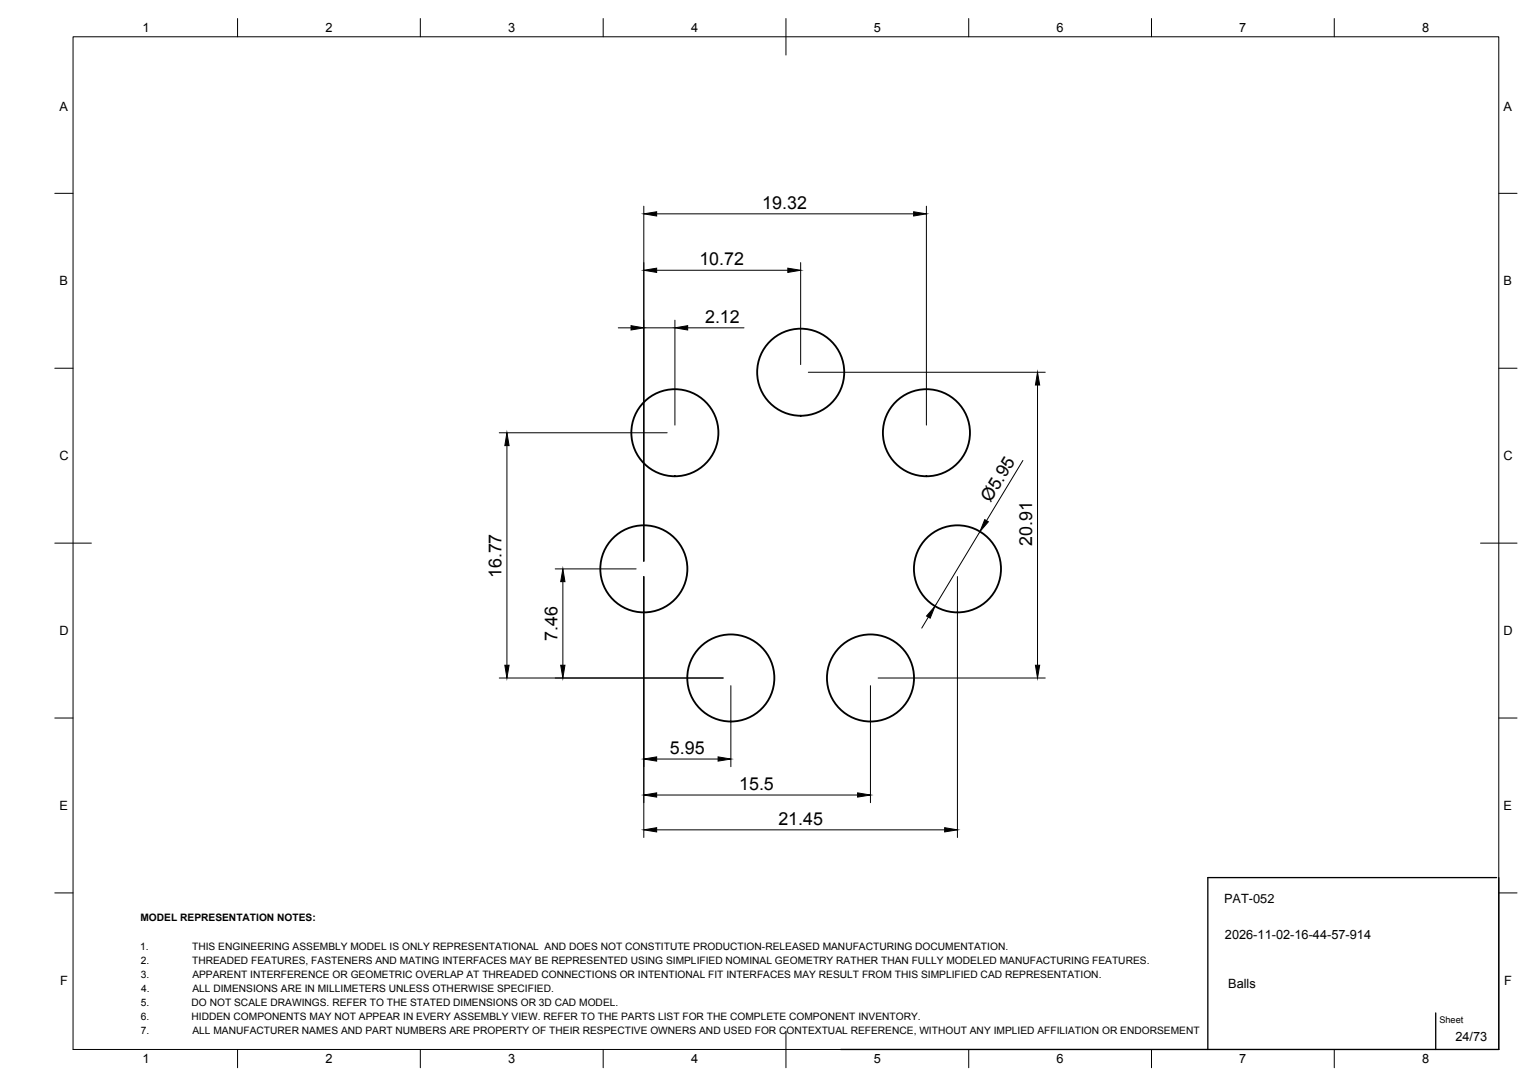
ISO-10303-21;
HEADER;
/* Generated by software containing ST-Developer
 * from STEP Tools, Inc. (www.steptools.com) 
 */

FILE_DESCRIPTION(
/* description */ ('Hand-crank gear train demonstrator'),
/* implementation_level */ '2;1');

FILE_NAME(
/* name */ 'Balls.step',
/* time_stamp */ '2026-10-28T03:22:13-07:00',
/* author */ (''),
/* organization */ (''),
/* preprocessor_version */ 'ST-DEVELOPER v20.2',
/* originating_system */ 'Autodesk Translation Framework v15.17.0.0',
/* authorisation */ '');

FILE_SCHEMA (('AUTOMOTIVE_DESIGN { 1 0 10303 214 3 1 1 }'));
ENDSEC;

DATA;
#10=MECHANICAL_DESIGN_GEOMETRIC_PRESENTATION_REPRESENTATION('',(#1202,#1203,#1204,#1205,#1206,#1207,#1208),#62758);
#991=SPHERICAL_SURFACE('',#17526,0.29765);
#992=SPHERICAL_SURFACE('',#17528,0.29765);
#993=SPHERICAL_SURFACE('',#17530,0.29765);
#994=SPHERICAL_SURFACE('',#17532,0.29765);
#995=SPHERICAL_SURFACE('',#17534,0.29765);
#996=SPHERICAL_SURFACE('',#17536,0.29765);
#997=SPHERICAL_SURFACE('',#17538,0.29765);
#1074=SHAPE_REPRESENTATION_RELATIONSHIP('SRR','None',#63047,#1138);
#1138=ADVANCED_BREP_SHAPE_REPRESENTATION('',(#1280,#1281,#1282,#1283,#1284,
#1285,#1286),#62701);
#1202=STYLED_ITEM('',(#63462),#1280);
#1203=STYLED_ITEM('',(#63462),#1281);
#1204=STYLED_ITEM('',(#63462),#1282);
#1205=STYLED_ITEM('',(#63462),#1283);
#1206=STYLED_ITEM('',(#63462),#1284);
#1207=STYLED_ITEM('',(#63462),#1285);
#1208=STYLED_ITEM('',(#63462),#1286);
#1280=MANIFOLD_SOLID_BREP('Body1',#16383);
#1281=MANIFOLD_SOLID_BREP('Body2',#16384);
#1282=MANIFOLD_SOLID_BREP('Body3',#16385);
#1283=MANIFOLD_SOLID_BREP('Body4',#16386);
#1284=MANIFOLD_SOLID_BREP('Body5',#16387);
#1285=MANIFOLD_SOLID_BREP('Body6',#16388);
#1286=MANIFOLD_SOLID_BREP('Body7',#16389);
#2277=FACE_OUTER_BOUND('',#3362,.T.);
#2278=FACE_OUTER_BOUND('',#3363,.T.);
#2279=FACE_OUTER_BOUND('',#3364,.T.);
#2280=FACE_OUTER_BOUND('',#3365,.T.);
#2281=FACE_OUTER_BOUND('',#3366,.T.);
#2282=FACE_OUTER_BOUND('',#3367,.T.);
#2283=FACE_OUTER_BOUND('',#3368,.T.);
#3362=EDGE_LOOP('',(#11523,#11524));
#3363=EDGE_LOOP('',(#11525,#11526));
#3364=EDGE_LOOP('',(#11527,#11528));
#3365=EDGE_LOOP('',(#11529,#11530));
#3366=EDGE_LOOP('',(#11531,#11532));
#3367=EDGE_LOOP('',(#11533,#11534));
#3368=EDGE_LOOP('',(#11535,#11536));
#6747=CIRCLE('',#17527,0.29765);
#6748=CIRCLE('',#17529,0.29765);
#6749=CIRCLE('',#17531,0.29765);
#6750=CIRCLE('',#17533,0.29765);
#6751=CIRCLE('',#17535,0.29765);
#6752=CIRCLE('',#17537,0.29765);
#6753=CIRCLE('',#17539,0.29765);
#7439=VERTEX_POINT('',#24052);
#7440=VERTEX_POINT('',#24053);
#7441=VERTEX_POINT('',#24056);
#7442=VERTEX_POINT('',#24057);
#7443=VERTEX_POINT('',#24060);
#7444=VERTEX_POINT('',#24061);
#7445=VERTEX_POINT('',#24064);
#7446=VERTEX_POINT('',#24065);
#7447=VERTEX_POINT('',#24068);
#7448=VERTEX_POINT('',#24069);
#7449=VERTEX_POINT('',#24072);
#7450=VERTEX_POINT('',#24073);
#7451=VERTEX_POINT('',#24076);
#7452=VERTEX_POINT('',#24077);
#9013=EDGE_CURVE('',#7439,#7440,#6747,.T.);
#9014=EDGE_CURVE('',#7441,#7442,#6748,.T.);
#9015=EDGE_CURVE('',#7443,#7444,#6749,.T.);
#9016=EDGE_CURVE('',#7445,#7446,#6750,.T.);
#9017=EDGE_CURVE('',#7447,#7448,#6751,.T.);
#9018=EDGE_CURVE('',#7449,#7450,#6752,.T.);
#9019=EDGE_CURVE('',#7451,#7452,#6753,.T.);
#11523=ORIENTED_EDGE('',*,*,#9013,.T.);
#11524=ORIENTED_EDGE('',*,*,#9013,.F.);
#11525=ORIENTED_EDGE('',*,*,#9014,.T.);
#11526=ORIENTED_EDGE('',*,*,#9014,.F.);
#11527=ORIENTED_EDGE('',*,*,#9015,.T.);
#11528=ORIENTED_EDGE('',*,*,#9015,.F.);
#11529=ORIENTED_EDGE('',*,*,#9016,.T.);
#11530=ORIENTED_EDGE('',*,*,#9016,.F.);
#11531=ORIENTED_EDGE('',*,*,#9017,.T.);
#11532=ORIENTED_EDGE('',*,*,#9017,.F.);
#11533=ORIENTED_EDGE('',*,*,#9018,.T.);
#11534=ORIENTED_EDGE('',*,*,#9018,.F.);
#11535=ORIENTED_EDGE('',*,*,#9019,.T.);
#11536=ORIENTED_EDGE('',*,*,#9019,.F.);
#15587=ADVANCED_FACE('',(#2277),#991,.T.);
#15588=ADVANCED_FACE('',(#2278),#992,.T.);
#15589=ADVANCED_FACE('',(#2279),#993,.T.);
#15590=ADVANCED_FACE('',(#2280),#994,.T.);
#15591=ADVANCED_FACE('',(#2281),#995,.T.);
#15592=ADVANCED_FACE('',(#2282),#996,.T.);
#15593=ADVANCED_FACE('',(#2283),#997,.T.);
#16383=CLOSED_SHELL('',(#15587));
#16384=CLOSED_SHELL('',(#15588));
#16385=CLOSED_SHELL('',(#15589));
#16386=CLOSED_SHELL('',(#15590));
#16387=CLOSED_SHELL('',(#15591));
#16388=CLOSED_SHELL('',(#15592));
#16389=CLOSED_SHELL('',(#15593));
#17525=AXIS2_PLACEMENT_3D('',#24050,#19712,#19713);
#17526=AXIS2_PLACEMENT_3D('',#24051,#19714,#19715);
#17527=AXIS2_PLACEMENT_3D('',#24054,#19716,#19717);
#17528=AXIS2_PLACEMENT_3D('',#24055,#19718,#19719);
#17529=AXIS2_PLACEMENT_3D('',#24058,#19720,#19721);
#17530=AXIS2_PLACEMENT_3D('',#24059,#19722,#19723);
#17531=AXIS2_PLACEMENT_3D('',#24062,#19724,#19725);
#17532=AXIS2_PLACEMENT_3D('',#24063,#19726,#19727);
#17533=AXIS2_PLACEMENT_3D('',#24066,#19728,#19729);
#17534=AXIS2_PLACEMENT_3D('',#24067,#19730,#19731);
#17535=AXIS2_PLACEMENT_3D('',#24070,#19732,#19733);
#17536=AXIS2_PLACEMENT_3D('',#24071,#19734,#19735);
#17537=AXIS2_PLACEMENT_3D('',#24074,#19736,#19737);
#17538=AXIS2_PLACEMENT_3D('',#24075,#19738,#19739);
#17539=AXIS2_PLACEMENT_3D('',#24078,#19740,#19741);
#19712=DIRECTION('axis',(0.,0.,1.));
#19713=DIRECTION('refdir',(1.,0.,0.));
#19714=DIRECTION('center_axis',(0.,0.,1.));
#19715=DIRECTION('ref_axis',(1.,0.,0.));
#19716=DIRECTION('center_axis',(1.22464679914735E-16,-1.,0.));
#19717=DIRECTION('ref_axis',(-1.,-1.22464679914735E-16,0.));
#19718=DIRECTION('center_axis',(0.78183148246803,0.,0.623489801858733));
#19719=DIRECTION('ref_axis',(0.623489801858734,0.,-0.78183148246803));
#19720=DIRECTION('center_axis',(7.63554790147315E-17,-1.,-9.57467422477103E-17));
#19721=DIRECTION('ref_axis',(-0.623489801858734,-1.22464679914735E-16,0.78183148246803));
#19722=DIRECTION('center_axis',(0.974927912181824,0.,-0.222520933956314));
#19723=DIRECTION('ref_axis',(-0.222520933956314,0.,-0.974927912181824));
#19724=DIRECTION('center_axis',(-2.7250954951288E-17,-1.,-1.19394234705288E-16));
#19725=DIRECTION('ref_axis',(0.222520933956314,-1.22464679914735E-16,0.974927912181824));
#19726=DIRECTION('center_axis',(0.433883739117558,0.,-0.900968867902419));
#19727=DIRECTION('ref_axis',(-0.900968867902419,0.,-0.433883739117558));
#19728=DIRECTION('center_axis',(-1.10336864020811E-16,-1.,-5.31354332312403E-17));
#19729=DIRECTION('ref_axis',(0.900968867902419,-1.22464679914735E-16,0.433883739117558));
#19730=DIRECTION('center_axis',(-0.433883739117558,0.,-0.900968867902419));
#19731=DIRECTION('ref_axis',(-0.900968867902419,0.,0.433883739117558));
#19732=DIRECTION('center_axis',(-1.10336864020811E-16,-1.,5.31354332312403E-17));
#19733=DIRECTION('ref_axis',(0.900968867902419,-1.22464679914735E-16,-0.433883739117558));
#19734=DIRECTION('center_axis',(-0.974927912181824,0.,-0.222520933956314));
#19735=DIRECTION('ref_axis',(-0.222520933956315,0.,0.974927912181824));
#19736=DIRECTION('center_axis',(-2.7250954951288E-17,-1.,1.19394234705288E-16));
#19737=DIRECTION('ref_axis',(0.222520933956315,-1.22464679914735E-16,-0.974927912181824));
#19738=DIRECTION('center_axis',(-0.78183148246803,0.,0.623489801858734));
#19739=DIRECTION('ref_axis',(0.623489801858733,0.,0.78183148246803));
#19740=DIRECTION('center_axis',(7.63554790147315E-17,-1.,9.57467422477103E-17));
#19741=DIRECTION('ref_axis',(-0.623489801858733,-1.22464679914735E-16,-0.78183148246803));
#24050=CARTESIAN_POINT('',(0.,0.,0.));
#24051=CARTESIAN_POINT('Origin',(1.1,0.,0.));
#24052=CARTESIAN_POINT('',(1.1,-2.23201749654651E-33,0.29765));
#24053=CARTESIAN_POINT('',(1.1,-2.23201749654651E-33,-0.29765));
#24054=CARTESIAN_POINT('Origin',(1.1,0.,0.));
#24055=CARTESIAN_POINT('Origin',(0.685838782044607,0.,-0.860014630714833));
#24056=CARTESIAN_POINT('',(0.918550922801216,-5.31350540756609E-33,-0.674432891191581));
#24057=CARTESIAN_POINT('',(0.453126641287998,8.49470414473068E-34,-1.04559637023808));
#24058=CARTESIAN_POINT('Origin',(0.685838782044607,0.,-0.860014630714833));
#24059=CARTESIAN_POINT('Origin',(-0.244773027351946,0.,-1.07242070340001));
#24060=CARTESIAN_POINT('',(0.0454142657089739,-2.23201749654651E-33,-1.1386540593921));
#24061=CARTESIAN_POINT('',(-0.534960320412865,-2.23201749654651E-33,-1.00618734740791));
#24062=CARTESIAN_POINT('Origin',(-0.244773027351946,0.,-1.07242070340001));
#24063=CARTESIAN_POINT('Origin',(-0.991065754692661,0.,-0.477272113029314));
#24064=CARTESIAN_POINT('',(-0.86192025974432,8.49470414473067E-34,-0.745445496560469));
#24065=CARTESIAN_POINT('',(-1.120211249641,-5.31350540756609E-33,-0.209098729498159));
#24066=CARTESIAN_POINT('Origin',(-0.991065754692661,0.,-0.477272113029314));
#24067=CARTESIAN_POINT('Origin',(-0.991065754692661,0.,0.477272113029314));
#24068=CARTESIAN_POINT('',(-1.120211249641,-2.23201749654651E-33,0.209098729498159));
#24069=CARTESIAN_POINT('',(-0.86192025974432,-2.23201749654651E-33,0.745445496560469));
#24070=CARTESIAN_POINT('Origin',(-0.991065754692661,0.,0.477272113029314));
#24071=CARTESIAN_POINT('Origin',(-0.244773027351946,0.,1.07242070340001));
#24072=CARTESIAN_POINT('',(-0.534960320412866,-2.23201749654651E-33,1.00618734740791));
#24073=CARTESIAN_POINT('',(0.0454142657089737,-2.23201749654651E-33,1.1386540593921));
#24074=CARTESIAN_POINT('Origin',(-0.244773027351946,0.,1.07242070340001));
#24075=CARTESIAN_POINT('Origin',(0.685838782044607,0.,0.860014630714833));
#24076=CARTESIAN_POINT('',(0.453126641287998,-2.23201749654651E-33,1.04559637023808));
#24077=CARTESIAN_POINT('',(0.918550922801216,-2.23201749654651E-33,0.674432891191581));
#24078=CARTESIAN_POINT('Origin',(0.685838782044607,0.,0.860014630714833));
#62627=UNCERTAINTY_MEASURE_WITH_UNIT(LENGTH_MEASURE(0.001),#62759,
'DISTANCE_ACCURACY_VALUE',
'Maximum model space distance between geometric entities at asserted c
onnectivities');
#62684=UNCERTAINTY_MEASURE_WITH_UNIT(LENGTH_MEASURE(0.001),#62759,
'DISTANCE_ACCURACY_VALUE',
'Maximum model space distance between geometric entities at asserted c
onnectivities');
#62701=(
GEOMETRIC_REPRESENTATION_CONTEXT(3)
GLOBAL_UNCERTAINTY_ASSIGNED_CONTEXT((#62627))
GLOBAL_UNIT_ASSIGNED_CONTEXT((#62759,#62761,#62762))
REPRESENTATION_CONTEXT('','3D')
);
#62758=(
GEOMETRIC_REPRESENTATION_CONTEXT(3)
GLOBAL_UNCERTAINTY_ASSIGNED_CONTEXT((#62684))
GLOBAL_UNIT_ASSIGNED_CONTEXT((#62759,#62761,#62762))
REPRESENTATION_CONTEXT('','3D')
);
#62759=(
LENGTH_UNIT()
NAMED_UNIT(*)
SI_UNIT(.CENTI.,.METRE.)
);
#62761=(
NAMED_UNIT(*)
PLANE_ANGLE_UNIT()
SI_UNIT($,.RADIAN.)
);
#62762=(
NAMED_UNIT(*)
SI_UNIT($,.STERADIAN.)
SOLID_ANGLE_UNIT()
);
#62779=SHAPE_DEFINITION_REPRESENTATION(#62852,#63047);
#62852=PRODUCT_DEFINITION_SHAPE('',$,#63121);
#63047=SHAPE_REPRESENTATION('',(#17525),#62701);
#63104=PRODUCT_DEFINITION_CONTEXT('part definition',#63325,'design');
#63121=PRODUCT_DEFINITION('Balls','Balls',#63194,#63104);
#63194=PRODUCT_DEFINITION_FORMATION('',$,#63343);
#63325=APPLICATION_CONTEXT(
'Core Data for Automotive Mechanical Design Process');
#63326=PRODUCT_CONTEXT('part definition',#63325,'mechanical');
#63343=PRODUCT('Balls','Balls','Balls',(#63326));
#63456=COLOUR_RGB('Grey',0.48,0.52,0.57);
#63457=FILL_AREA_STYLE_COLOUR('',#63456);
#63458=FILL_AREA_STYLE('',(#63457));
#63459=SURFACE_STYLE_FILL_AREA(#63458);
#63460=SURFACE_SIDE_STYLE('',(#63459));
#63461=SURFACE_STYLE_USAGE(.BOTH.,#63460);
#63462=PRESENTATION_STYLE_ASSIGNMENT((#63461));
ENDSEC;
END-ISO-10303-21;
